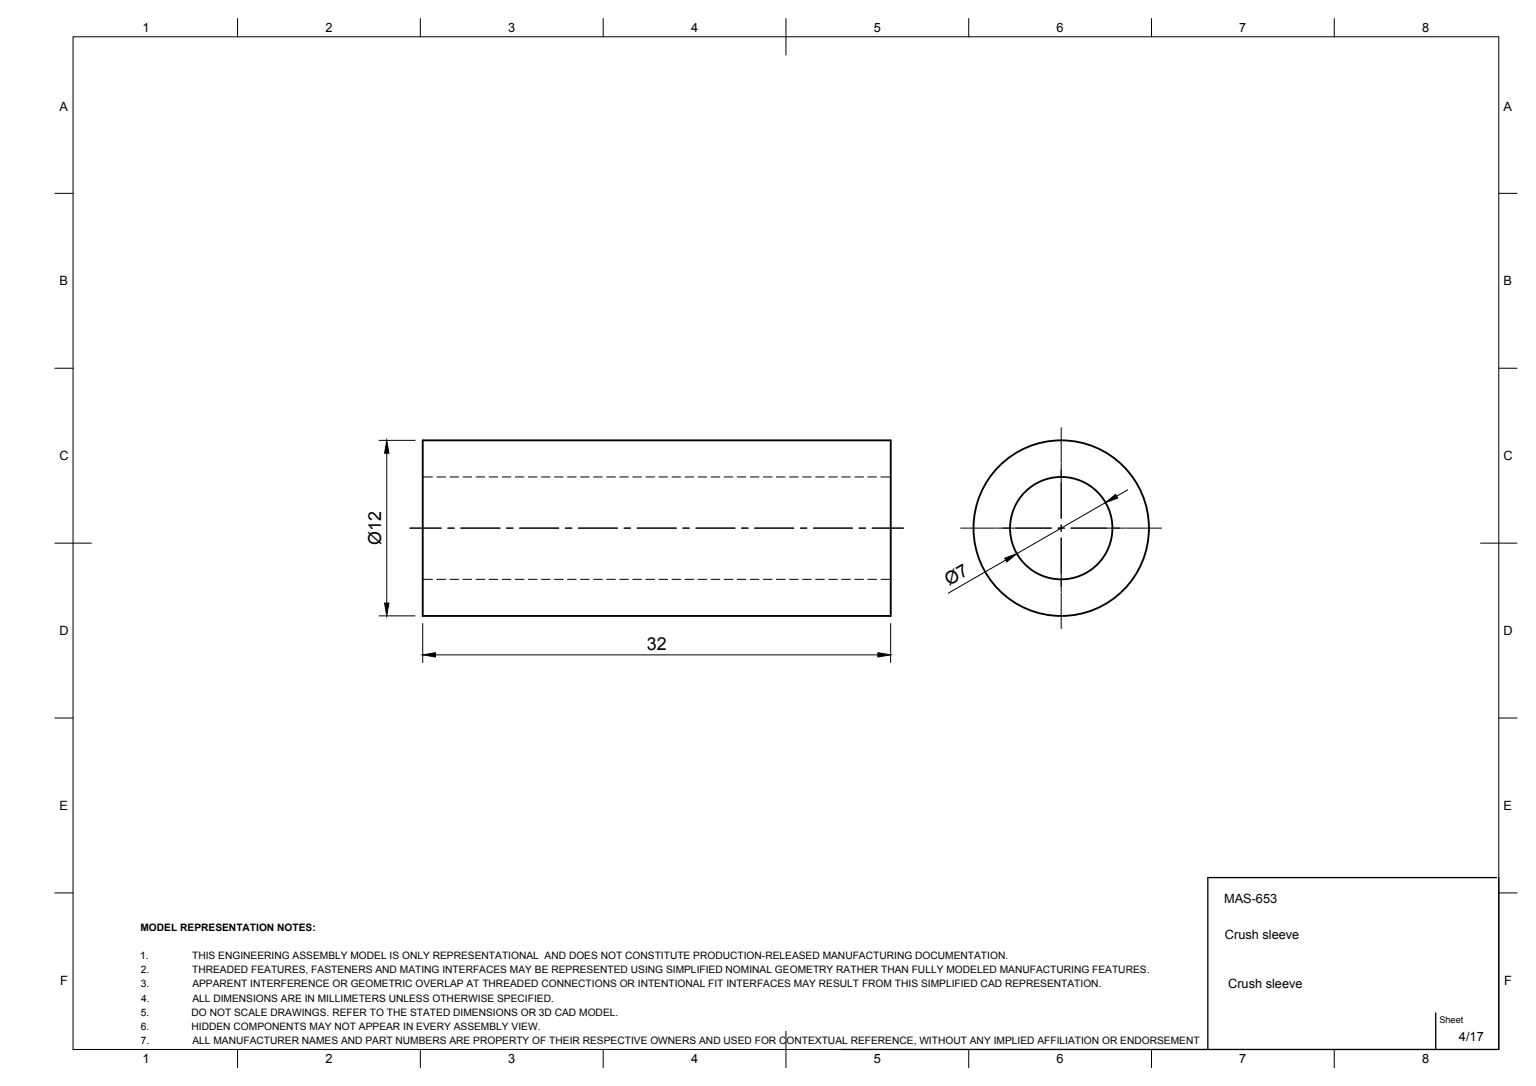
ISO-10303-21;
HEADER;
/* Generated by software containing ST-Developer
 * from STEP Tools, Inc. (www.steptools.com) 
 */

FILE_DESCRIPTION(
/* description */ ('Independent compact industrial fixture table, bolted aluminum worktop
 on connected adjustable support base. Whole-mm nominal dimensions. No
 load rating assigned.'),
/* implementation_level */ '2;1');

FILE_NAME(
/* name */ 'Crush sleeve.step',
/* time_stamp */ '2026-11-07T17:47:58-08:00',
/* author */ (''),
/* organization */ (''),
/* preprocessor_version */ 'ST-DEVELOPER v20.2',
/* originating_system */ 'Autodesk Translation Framework v15.17.0.0',
/* authorisation */ '');

FILE_SCHEMA (('AUTOMOTIVE_DESIGN { 1 0 10303 214 3 1 1 }'));
ENDSEC;

DATA;
#10=MECHANICAL_DESIGN_GEOMETRIC_PRESENTATION_REPRESENTATION('',(#2267),#97475);
#2229=SHAPE_REPRESENTATION_RELATIONSHIP('SRR','None',#97623,#2248);
#2248=ADVANCED_BREP_SHAPE_REPRESENTATION('',(#2286),#97473);
#2267=STYLED_ITEM('',(#97722),#2286);
#2286=MANIFOLD_SOLID_BREP('Body1',#21828);
#2375=FACE_BOUND('',#4927,.T.);
#2376=FACE_BOUND('',#4929,.T.);
#2533=PLANE('',#23452);
#2534=PLANE('',#23453);
#3683=FACE_OUTER_BOUND('',#4924,.T.);
#3684=FACE_OUTER_BOUND('',#4925,.T.);
#3685=FACE_OUTER_BOUND('',#4926,.T.);
#3686=FACE_OUTER_BOUND('',#4928,.T.);
#4924=EDGE_LOOP('',(#19686,#19687,#19688,#19689));
#4925=EDGE_LOOP('',(#19690,#19691,#19692,#19693));
#4926=EDGE_LOOP('',(#19694));
#4927=EDGE_LOOP('',(#19695));
#4928=EDGE_LOOP('',(#19696));
#4929=EDGE_LOOP('',(#19697));
#6146=LINE('',#97366,#7360);
#6147=LINE('',#97372,#7361);
#7360=VECTOR('',#27528,3.5);
#7361=VECTOR('',#27535,6.);
#7605=CIRCLE('',#23447,3.5);
#7606=CIRCLE('',#23448,3.5);
#7607=CIRCLE('',#23450,6.);
#7608=CIRCLE('',#23451,6.);
#9805=VERTEX_POINT('',#97363);
#9806=VERTEX_POINT('',#97365);
#9807=VERTEX_POINT('',#97369);
#9808=VERTEX_POINT('',#97371);
#13100=EDGE_CURVE('',#9805,#9805,#7605,.T.);
#13101=EDGE_CURVE('',#9805,#9806,#6146,.T.);
#13102=EDGE_CURVE('',#9806,#9806,#7606,.T.);
#13103=EDGE_CURVE('',#9807,#9807,#7607,.T.);
#13104=EDGE_CURVE('',#9807,#9808,#6147,.T.);
#13105=EDGE_CURVE('',#9808,#9808,#7608,.T.);
#19686=ORIENTED_EDGE('',*,*,#13100,.F.);
#19687=ORIENTED_EDGE('',*,*,#13101,.T.);
#19688=ORIENTED_EDGE('',*,*,#13102,.T.);
#19689=ORIENTED_EDGE('',*,*,#13101,.F.);
#19690=ORIENTED_EDGE('',*,*,#13103,.F.);
#19691=ORIENTED_EDGE('',*,*,#13104,.T.);
#19692=ORIENTED_EDGE('',*,*,#13105,.T.);
#19693=ORIENTED_EDGE('',*,*,#13104,.F.);
#19694=ORIENTED_EDGE('',*,*,#13103,.T.);
#19695=ORIENTED_EDGE('',*,*,#13100,.T.);
#19696=ORIENTED_EDGE('',*,*,#13105,.F.);
#19697=ORIENTED_EDGE('',*,*,#13102,.F.);
#20653=CYLINDRICAL_SURFACE('',#23446,3.5);
#20654=CYLINDRICAL_SURFACE('',#23449,6.);
#21803=ADVANCED_FACE('',(#3683),#20653,.F.);
#21804=ADVANCED_FACE('',(#3684),#20654,.T.);
#21805=ADVANCED_FACE('',(#3685,#2375),#2533,.T.);
#21806=ADVANCED_FACE('',(#3686,#2376),#2534,.F.);
#21828=CLOSED_SHELL('',(#21803,#21804,#21805,#21806));
#23445=AXIS2_PLACEMENT_3D('',#97361,#27522,#27523);
#23446=AXIS2_PLACEMENT_3D('',#97362,#27524,#27525);
#23447=AXIS2_PLACEMENT_3D('',#97364,#27526,#27527);
#23448=AXIS2_PLACEMENT_3D('',#97367,#27529,#27530);
#23449=AXIS2_PLACEMENT_3D('',#97368,#27531,#27532);
#23450=AXIS2_PLACEMENT_3D('',#97370,#27533,#27534);
#23451=AXIS2_PLACEMENT_3D('',#97373,#27536,#27537);
#23452=AXIS2_PLACEMENT_3D('',#97374,#27538,#27539);
#23453=AXIS2_PLACEMENT_3D('',#97375,#27540,#27541);
#27522=DIRECTION('axis',(0.,0.,1.));
#27523=DIRECTION('refdir',(1.,0.,0.));
#27524=DIRECTION('center_axis',(0.,0.,1.));
#27525=DIRECTION('ref_axis',(1.,0.,0.));
#27526=DIRECTION('center_axis',(0.,0.,-1.));
#27527=DIRECTION('ref_axis',(1.,0.,0.));
#27528=DIRECTION('',(0.,0.,-1.));
#27529=DIRECTION('center_axis',(0.,0.,-1.));
#27530=DIRECTION('ref_axis',(1.,0.,0.));
#27531=DIRECTION('center_axis',(0.,0.,1.));
#27532=DIRECTION('ref_axis',(1.,0.,0.));
#27533=DIRECTION('center_axis',(0.,0.,1.));
#27534=DIRECTION('ref_axis',(1.,0.,0.));
#27535=DIRECTION('',(0.,0.,-1.));
#27536=DIRECTION('center_axis',(0.,0.,1.));
#27537=DIRECTION('ref_axis',(1.,0.,0.));
#27538=DIRECTION('center_axis',(0.,0.,1.));
#27539=DIRECTION('ref_axis',(1.,0.,0.));
#27540=DIRECTION('center_axis',(0.,0.,1.));
#27541=DIRECTION('ref_axis',(1.,0.,0.));
#97361=CARTESIAN_POINT('',(0.,0.,0.));
#97362=CARTESIAN_POINT('Origin',(0.,0.,0.));
#97363=CARTESIAN_POINT('',(-3.5,-4.28626379701574E-16,32.));
#97364=CARTESIAN_POINT('Origin',(0.,0.,32.));
#97365=CARTESIAN_POINT('',(-3.5,-4.28626379701574E-16,0.));
#97366=CARTESIAN_POINT('',(-3.5,-4.28626379701574E-16,0.));
#97367=CARTESIAN_POINT('Origin',(0.,0.,0.));
#97368=CARTESIAN_POINT('Origin',(0.,0.,0.));
#97369=CARTESIAN_POINT('',(-6.,-7.34788079488412E-16,32.));
#97370=CARTESIAN_POINT('Origin',(0.,0.,32.));
#97371=CARTESIAN_POINT('',(-6.,-7.34788079488412E-16,0.));
#97372=CARTESIAN_POINT('',(-6.,-7.34788079488412E-16,0.));
#97373=CARTESIAN_POINT('Origin',(0.,0.,0.));
#97374=CARTESIAN_POINT('Origin',(0.,0.,32.));
#97375=CARTESIAN_POINT('Origin',(0.,0.,0.));
#97450=UNCERTAINTY_MEASURE_WITH_UNIT(LENGTH_MEASURE(0.01),#97476,
'DISTANCE_ACCURACY_VALUE',
'Maximum model space distance between geometric entities at asserted c
onnectivities');
#97452=UNCERTAINTY_MEASURE_WITH_UNIT(LENGTH_MEASURE(0.01),#97476,
'DISTANCE_ACCURACY_VALUE',
'Maximum model space distance between geometric entities at asserted c
onnectivities');
#97473=(
GEOMETRIC_REPRESENTATION_CONTEXT(3)
GLOBAL_UNCERTAINTY_ASSIGNED_CONTEXT((#97450))
GLOBAL_UNIT_ASSIGNED_CONTEXT((#97476,#97478,#97479))
REPRESENTATION_CONTEXT('','3D')
);
#97475=(
GEOMETRIC_REPRESENTATION_CONTEXT(3)
GLOBAL_UNCERTAINTY_ASSIGNED_CONTEXT((#97452))
GLOBAL_UNIT_ASSIGNED_CONTEXT((#97476,#97478,#97479))
REPRESENTATION_CONTEXT('','3D')
);
#97476=(
LENGTH_UNIT()
NAMED_UNIT(*)
SI_UNIT(.MILLI.,.METRE.)
);
#97478=(
NAMED_UNIT(*)
PLANE_ANGLE_UNIT()
SI_UNIT($,.RADIAN.)
);
#97479=(
NAMED_UNIT(*)
SI_UNIT($,.STERADIAN.)
SOLID_ANGLE_UNIT()
);
#97500=SHAPE_DEFINITION_REPRESENTATION(#97562,#97623);
#97562=PRODUCT_DEFINITION_SHAPE('',$,#97646);
#97623=SHAPE_REPRESENTATION('',(#23445),#97473);
#97625=PRODUCT_DEFINITION_CONTEXT('part definition',#97693,'design');
#97646=PRODUCT_DEFINITION('Crush sleeve','Crush sleeve',#97668,#97625);
#97668=PRODUCT_DEFINITION_FORMATION('',$,#97715);
#97693=APPLICATION_CONTEXT(
'Core Data for Automotive Mechanical Design Process');
#97694=PRODUCT_CONTEXT('part definition',#97693,'mechanical');
#97715=PRODUCT('Crush sleeve','Crush sleeve',
'Steel compression sleeve inside the hollow frame tube; protects tube 
walls when worktop fasteners are tightened.',(#97694));
#97722=PRESENTATION_STYLE_ASSIGNMENT((#97729));
#97729=SURFACE_STYLE_USAGE(.BOTH.,#97736);
#97736=SURFACE_SIDE_STYLE('',(#97743));
#97743=SURFACE_STYLE_FILL_AREA(#97750);
#97750=FILL_AREA_STYLE('Gray',(#97757));
#97757=FILL_AREA_STYLE_COLOUR('Gray',#97764);
#97764=COLOUR_RGB('Gray',0.407843137254902,0.447058823529412,0.498039215686275);
ENDSEC;
END-ISO-10303-21;
